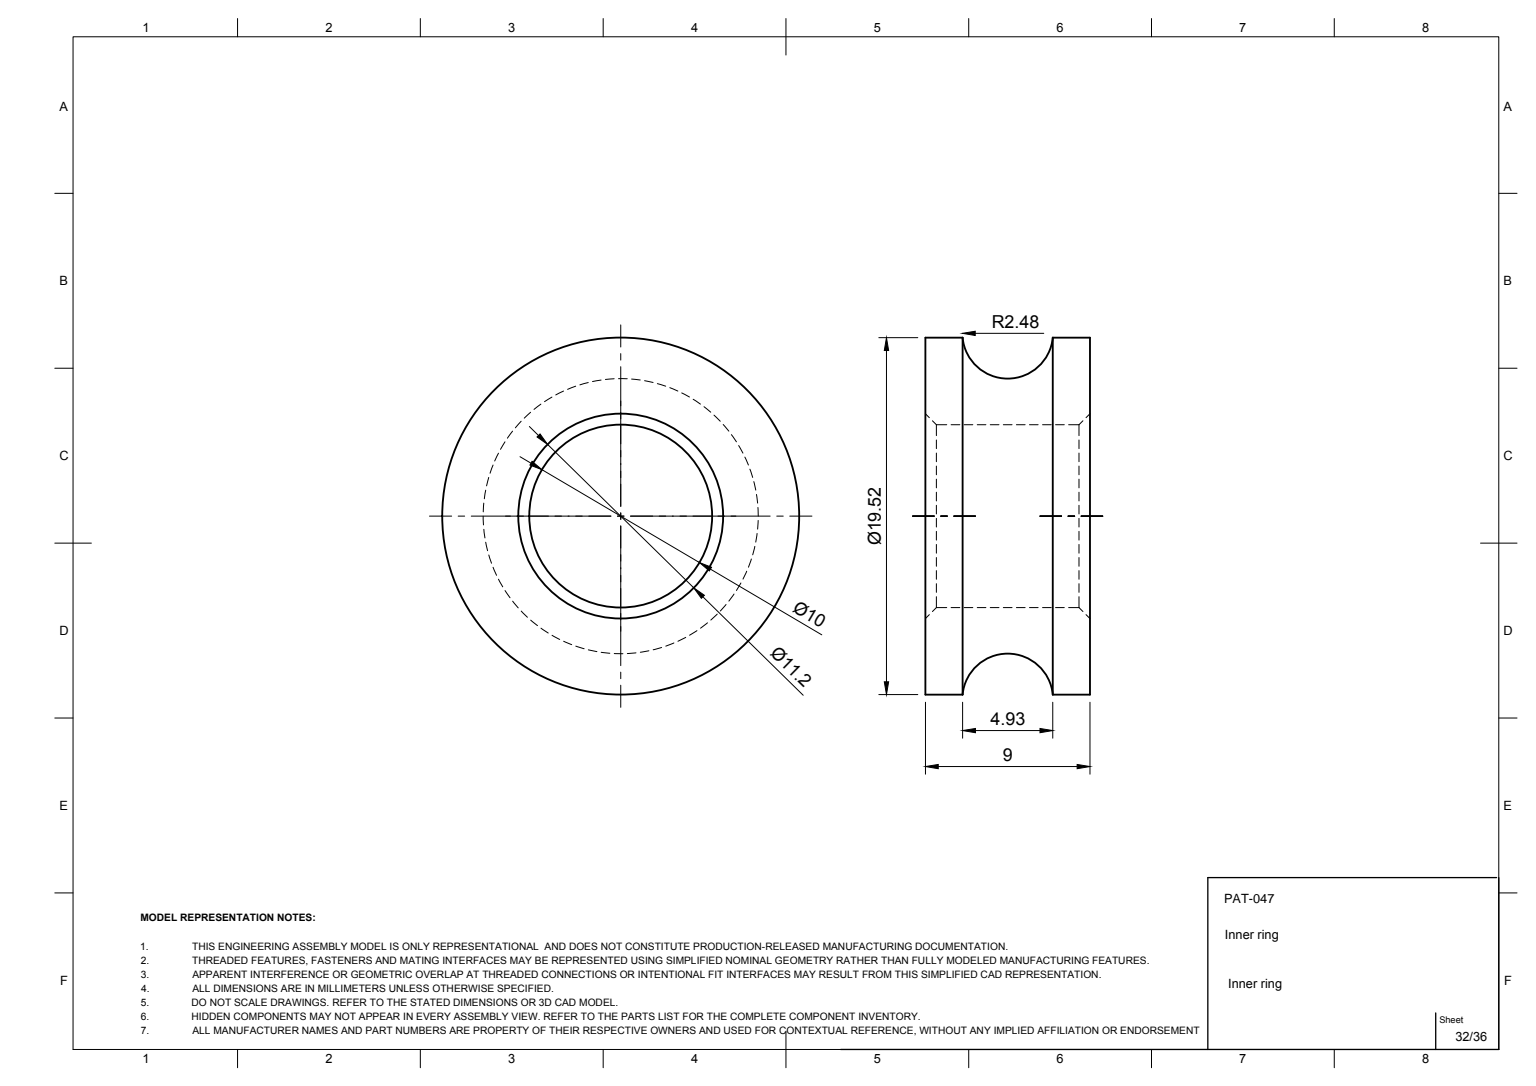
ISO-10303-21;
HEADER;
/* Generated by software containing ST-Developer
 * from STEP Tools, Inc. (www.steptools.com) 
 */

FILE_DESCRIPTION(
/* description */ ('Gravity roller conveyor section'),
/* implementation_level */ '2;1');

FILE_NAME(
/* name */ 'Inner ring.step',
/* time_stamp */ '2026-11-02T07:43:02-08:00',
/* author */ (''),
/* organization */ (''),
/* preprocessor_version */ 'ST-DEVELOPER v20.2',
/* originating_system */ 'Autodesk Translation Framework v15.17.0.0',
/* authorisation */ '');

FILE_SCHEMA (('AUTOMOTIVE_DESIGN { 1 0 10303 214 3 1 1 }'));
ENDSEC;

DATA;
#10=MECHANICAL_DESIGN_GEOMETRIC_PRESENTATION_REPRESENTATION('',(#552),#13821);
#405=TOROIDAL_SURFACE('',#8485,1.,0.247676);
#415=CONICAL_SURFACE('',#8496,0.53,0.785398163397448);
#416=CONICAL_SURFACE('',#8503,0.53,0.785398163397448);
#484=SHAPE_REPRESENTATION_RELATIONSHIP('SRR','None',#14023,#518);
#518=ADVANCED_BREP_SHAPE_REPRESENTATION('',(#592),#13810);
#552=STYLED_ITEM('',(#14191),#592);
#592=MANIFOLD_SOLID_BREP('Body1',#7652);
#678=FACE_BOUND('',#1801,.T.);
#679=FACE_BOUND('',#1804,.T.);
#943=PLANE('',#8498);
#944=PLANE('',#8501);
#1308=FACE_OUTER_BOUND('',#1796,.T.);
#1309=FACE_OUTER_BOUND('',#1797,.T.);
#1310=FACE_OUTER_BOUND('',#1798,.T.);
#1311=FACE_OUTER_BOUND('',#1799,.T.);
#1312=FACE_OUTER_BOUND('',#1800,.T.);
#1313=FACE_OUTER_BOUND('',#1802,.T.);
#1314=FACE_OUTER_BOUND('',#1803,.T.);
#1315=FACE_OUTER_BOUND('',#1805,.T.);
#1796=EDGE_LOOP('',(#6642,#6643,#6644,#6645,#6646,#6647));
#1797=EDGE_LOOP('',(#6648,#6649,#6650,#6651,#6652));
#1798=EDGE_LOOP('',(#6653,#6654,#6655,#6656));
#1799=EDGE_LOOP('',(#6657,#6658,#6659,#6660));
#1800=EDGE_LOOP('',(#6661));
#1801=EDGE_LOOP('',(#6662));
#1802=EDGE_LOOP('',(#6663,#6664,#6665,#6666,#6667));
#1803=EDGE_LOOP('',(#6668));
#1804=EDGE_LOOP('',(#6669));
#1805=EDGE_LOOP('',(#6670,#6671,#6672,#6673));
#2540=LINE('',#12782,#3258);
#2541=LINE('',#12788,#3259);
#2542=LINE('',#12792,#3260);
#2543=LINE('',#12798,#3261);
#2544=LINE('',#12803,#3262);
#3258=VECTOR('',#10307,0.976185);
#3259=VECTOR('',#10314,0.5);
#3260=VECTOR('',#10319,0.53);
#3261=VECTOR('',#10328,0.976185);
#3262=VECTOR('',#10335,0.53);
#3482=CIRCLE('',#8486,0.976185);
#3483=CIRCLE('',#8487,0.976185);
#3484=CIRCLE('',#8488,0.247676);
#3485=CIRCLE('',#8489,0.976185);
#3486=CIRCLE('',#8490,0.976185);
#3487=CIRCLE('',#8492,0.976185);
#3488=CIRCLE('',#8494,0.5);
#3489=CIRCLE('',#8495,0.5);
#3490=CIRCLE('',#8497,0.56);
#3491=CIRCLE('',#8500,0.976185);
#3492=CIRCLE('',#8502,0.56);
#4068=VERTEX_POINT('',#12771);
#4069=VERTEX_POINT('',#12772);
#4070=VERTEX_POINT('',#12775);
#4071=VERTEX_POINT('',#12777);
#4072=VERTEX_POINT('',#12781);
#4073=VERTEX_POINT('',#12785);
#4074=VERTEX_POINT('',#12787);
#4075=VERTEX_POINT('',#12791);
#4076=VERTEX_POINT('',#12796);
#4077=VERTEX_POINT('',#12800);
#4958=EDGE_CURVE('',#4068,#4069,#3482,.T.);
#4959=EDGE_CURVE('',#4069,#4068,#3483,.T.);
#4960=EDGE_CURVE('',#4069,#4070,#3484,.T.);
#4961=EDGE_CURVE('',#4071,#4070,#3485,.T.);
#4962=EDGE_CURVE('',#4070,#4071,#3486,.T.);
#4963=EDGE_CURVE('',#4071,#4072,#2540,.T.);
#4964=EDGE_CURVE('',#4072,#4072,#3487,.T.);
#4965=EDGE_CURVE('',#4073,#4073,#3488,.T.);
#4966=EDGE_CURVE('',#4073,#4074,#2541,.T.);
#4967=EDGE_CURVE('',#4074,#4074,#3489,.T.);
#4968=EDGE_CURVE('',#4074,#4075,#2542,.T.);
#4969=EDGE_CURVE('',#4075,#4075,#3490,.T.);
#4970=EDGE_CURVE('',#4076,#4076,#3491,.T.);
#4971=EDGE_CURVE('',#4076,#4068,#2543,.T.);
#4972=EDGE_CURVE('',#4077,#4077,#3492,.T.);
#4973=EDGE_CURVE('',#4077,#4073,#2544,.T.);
#6642=ORIENTED_EDGE('',*,*,#4958,.F.);
#6643=ORIENTED_EDGE('',*,*,#4959,.F.);
#6644=ORIENTED_EDGE('',*,*,#4960,.T.);
#6645=ORIENTED_EDGE('',*,*,#4961,.F.);
#6646=ORIENTED_EDGE('',*,*,#4962,.F.);
#6647=ORIENTED_EDGE('',*,*,#4960,.F.);
#6648=ORIENTED_EDGE('',*,*,#4961,.T.);
#6649=ORIENTED_EDGE('',*,*,#4962,.T.);
#6650=ORIENTED_EDGE('',*,*,#4963,.T.);
#6651=ORIENTED_EDGE('',*,*,#4964,.T.);
#6652=ORIENTED_EDGE('',*,*,#4963,.F.);
#6653=ORIENTED_EDGE('',*,*,#4965,.T.);
#6654=ORIENTED_EDGE('',*,*,#4966,.T.);
#6655=ORIENTED_EDGE('',*,*,#4967,.F.);
#6656=ORIENTED_EDGE('',*,*,#4966,.F.);
#6657=ORIENTED_EDGE('',*,*,#4967,.T.);
#6658=ORIENTED_EDGE('',*,*,#4968,.T.);
#6659=ORIENTED_EDGE('',*,*,#4969,.F.);
#6660=ORIENTED_EDGE('',*,*,#4968,.F.);
#6661=ORIENTED_EDGE('',*,*,#4964,.F.);
#6662=ORIENTED_EDGE('',*,*,#4969,.T.);
#6663=ORIENTED_EDGE('',*,*,#4970,.F.);
#6664=ORIENTED_EDGE('',*,*,#4971,.T.);
#6665=ORIENTED_EDGE('',*,*,#4958,.T.);
#6666=ORIENTED_EDGE('',*,*,#4959,.T.);
#6667=ORIENTED_EDGE('',*,*,#4971,.F.);
#6668=ORIENTED_EDGE('',*,*,#4970,.T.);
#6669=ORIENTED_EDGE('',*,*,#4972,.F.);
#6670=ORIENTED_EDGE('',*,*,#4972,.T.);
#6671=ORIENTED_EDGE('',*,*,#4973,.T.);
#6672=ORIENTED_EDGE('',*,*,#4965,.F.);
#6673=ORIENTED_EDGE('',*,*,#4973,.F.);
#7182=CYLINDRICAL_SURFACE('',#8491,0.976185);
#7183=CYLINDRICAL_SURFACE('',#8493,0.5);
#7184=CYLINDRICAL_SURFACE('',#8499,0.976185);
#7509=ADVANCED_FACE('',(#1308),#405,.F.);
#7510=ADVANCED_FACE('',(#1309),#7182,.T.);
#7511=ADVANCED_FACE('',(#1310),#7183,.F.);
#7512=ADVANCED_FACE('',(#1311),#415,.F.);
#7513=ADVANCED_FACE('',(#1312,#678),#943,.T.);
#7514=ADVANCED_FACE('',(#1313),#7184,.T.);
#7515=ADVANCED_FACE('',(#1314,#679),#944,.T.);
#7516=ADVANCED_FACE('',(#1315),#416,.F.);
#7652=CLOSED_SHELL('',(#7509,#7510,#7511,#7512,#7513,#7514,#7515,#7516));
#8484=AXIS2_PLACEMENT_3D('',#12769,#10291,#10292);
#8485=AXIS2_PLACEMENT_3D('',#12770,#10293,#10294);
#8486=AXIS2_PLACEMENT_3D('',#12773,#10295,#10296);
#8487=AXIS2_PLACEMENT_3D('',#12774,#10297,#10298);
#8488=AXIS2_PLACEMENT_3D('',#12776,#10299,#10300);
#8489=AXIS2_PLACEMENT_3D('',#12778,#10301,#10302);
#8490=AXIS2_PLACEMENT_3D('',#12779,#10303,#10304);
#8491=AXIS2_PLACEMENT_3D('',#12780,#10305,#10306);
#8492=AXIS2_PLACEMENT_3D('',#12783,#10308,#10309);
#8493=AXIS2_PLACEMENT_3D('',#12784,#10310,#10311);
#8494=AXIS2_PLACEMENT_3D('',#12786,#10312,#10313);
#8495=AXIS2_PLACEMENT_3D('',#12789,#10315,#10316);
#8496=AXIS2_PLACEMENT_3D('',#12790,#10317,#10318);
#8497=AXIS2_PLACEMENT_3D('',#12793,#10320,#10321);
#8498=AXIS2_PLACEMENT_3D('',#12794,#10322,#10323);
#8499=AXIS2_PLACEMENT_3D('',#12795,#10324,#10325);
#8500=AXIS2_PLACEMENT_3D('',#12797,#10326,#10327);
#8501=AXIS2_PLACEMENT_3D('',#12799,#10329,#10330);
#8502=AXIS2_PLACEMENT_3D('',#12801,#10331,#10332);
#8503=AXIS2_PLACEMENT_3D('',#12802,#10333,#10334);
#10291=DIRECTION('axis',(0.,0.,1.));
#10292=DIRECTION('refdir',(1.,0.,0.));
#10293=DIRECTION('center_axis',(0.,-1.,0.));
#10294=DIRECTION('ref_axis',(0.,0.,-1.));
#10295=DIRECTION('center_axis',(0.,-1.,0.));
#10296=DIRECTION('ref_axis',(1.,0.,0.));
#10297=DIRECTION('center_axis',(0.,-1.,0.));
#10298=DIRECTION('ref_axis',(1.,0.,0.));
#10299=DIRECTION('center_axis',(1.,0.,1.22464679914735E-16));
#10300=DIRECTION('ref_axis',(-1.22464679914735E-16,0.,1.));
#10301=DIRECTION('center_axis',(0.,1.,0.));
#10302=DIRECTION('ref_axis',(1.,0.,0.));
#10303=DIRECTION('center_axis',(0.,1.,0.));
#10304=DIRECTION('ref_axis',(1.,0.,0.));
#10305=DIRECTION('center_axis',(0.,-1.,0.));
#10306=DIRECTION('ref_axis',(1.,0.,0.));
#10307=DIRECTION('',(0.,1.,0.));
#10308=DIRECTION('center_axis',(0.,-1.,0.));
#10309=DIRECTION('ref_axis',(1.,0.,0.));
#10310=DIRECTION('center_axis',(0.,-1.,0.));
#10311=DIRECTION('ref_axis',(1.,0.,0.));
#10312=DIRECTION('center_axis',(0.,-1.,0.));
#10313=DIRECTION('ref_axis',(1.,0.,0.));
#10314=DIRECTION('',(0.,1.,0.));
#10315=DIRECTION('center_axis',(0.,-1.,0.));
#10316=DIRECTION('ref_axis',(1.,0.,0.));
#10317=DIRECTION('center_axis',(0.,1.,0.));
#10318=DIRECTION('ref_axis',(1.,0.,0.));
#10319=DIRECTION('',(-0.707106781186547,0.707106781186548,-8.65956056235493E-17));
#10320=DIRECTION('center_axis',(0.,-1.,0.));
#10321=DIRECTION('ref_axis',(1.,0.,0.));
#10322=DIRECTION('center_axis',(0.,1.,0.));
#10323=DIRECTION('ref_axis',(0.,0.,1.));
#10324=DIRECTION('center_axis',(0.,-1.,0.));
#10325=DIRECTION('ref_axis',(1.,0.,0.));
#10326=DIRECTION('center_axis',(0.,-1.,0.));
#10327=DIRECTION('ref_axis',(1.,0.,0.));
#10328=DIRECTION('',(0.,1.,0.));
#10329=DIRECTION('center_axis',(0.,-1.,0.));
#10330=DIRECTION('ref_axis',(0.,0.,-1.));
#10331=DIRECTION('center_axis',(0.,-1.,0.));
#10332=DIRECTION('ref_axis',(1.,0.,0.));
#10333=DIRECTION('center_axis',(0.,-1.,0.));
#10334=DIRECTION('ref_axis',(1.,0.,0.));
#10335=DIRECTION('',(0.707106781186547,0.707106781186548,8.65956056235493E-17));
#12769=CARTESIAN_POINT('',(0.,0.,0.));
#12770=CARTESIAN_POINT('Origin',(0.,0.,0.));
#12771=CARTESIAN_POINT('',(-0.976185,-0.246528389340863,-1.19548183562566E-16));
#12772=CARTESIAN_POINT('',(-1.19548183562566E-16,-0.246528389340863,0.976185));
#12773=CARTESIAN_POINT('Origin',(0.,-0.246528389340863,0.));
#12774=CARTESIAN_POINT('Origin',(0.,-0.246528389340863,0.));
#12775=CARTESIAN_POINT('',(-1.19548183562566E-16,0.246528389340863,0.976185));
#12776=CARTESIAN_POINT('Origin',(-1.22464679914735E-16,0.,1.));
#12777=CARTESIAN_POINT('',(-0.976185,0.246528389340863,1.19548183562566E-16));
#12778=CARTESIAN_POINT('Origin',(0.,0.246528389340863,0.));
#12779=CARTESIAN_POINT('Origin',(0.,0.246528389340863,0.));
#12780=CARTESIAN_POINT('Origin',(0.,0.,0.));
#12781=CARTESIAN_POINT('',(-0.976185,0.45,-1.19548183562566E-16));
#12782=CARTESIAN_POINT('',(-0.976185,0.,-1.19548183562566E-16));
#12783=CARTESIAN_POINT('Origin',(0.,0.45,0.));
#12784=CARTESIAN_POINT('Origin',(0.,0.,0.));
#12785=CARTESIAN_POINT('',(-0.5,-0.39,-6.12323399573677E-17));
#12786=CARTESIAN_POINT('Origin',(0.,-0.39,0.));
#12787=CARTESIAN_POINT('',(-0.5,0.39,-6.12323399573677E-17));
#12788=CARTESIAN_POINT('',(-0.5,0.,-6.12323399573677E-17));
#12789=CARTESIAN_POINT('Origin',(0.,0.39,0.));
#12790=CARTESIAN_POINT('Origin',(0.,0.42,0.));
#12791=CARTESIAN_POINT('',(-0.56,0.45,-6.85802207522518E-17));
#12792=CARTESIAN_POINT('',(-0.53,0.42,-6.49062803548097E-17));
#12793=CARTESIAN_POINT('Origin',(0.,0.45,0.));
#12794=CARTESIAN_POINT('Origin',(0.976185,0.45,0.));
#12795=CARTESIAN_POINT('Origin',(0.,0.,0.));
#12796=CARTESIAN_POINT('',(-0.976185,-0.45,-1.19548183562566E-16));
#12797=CARTESIAN_POINT('Origin',(0.,-0.45,0.));
#12798=CARTESIAN_POINT('',(-0.976185,0.,-1.19548183562566E-16));
#12799=CARTESIAN_POINT('Origin',(0.56,-0.45,0.));
#12800=CARTESIAN_POINT('',(-0.56,-0.45,-6.85802207522518E-17));
#12801=CARTESIAN_POINT('Origin',(0.,-0.45,0.));
#12802=CARTESIAN_POINT('Origin',(0.,-0.42,0.));
#12803=CARTESIAN_POINT('',(-0.53,-0.42,-6.49062803548097E-17));
#13771=UNCERTAINTY_MEASURE_WITH_UNIT(LENGTH_MEASURE(0.001),#13822,
'DISTANCE_ACCURACY_VALUE',
'Maximum model space distance between geometric entities at asserted c
onnectivities');
#13782=UNCERTAINTY_MEASURE_WITH_UNIT(LENGTH_MEASURE(0.001),#13822,
'DISTANCE_ACCURACY_VALUE',
'Maximum model space distance between geometric entities at asserted c
onnectivities');
#13810=(
GEOMETRIC_REPRESENTATION_CONTEXT(3)
GLOBAL_UNCERTAINTY_ASSIGNED_CONTEXT((#13771))
GLOBAL_UNIT_ASSIGNED_CONTEXT((#13822,#13824,#13825))
REPRESENTATION_CONTEXT('','3D')
);
#13821=(
GEOMETRIC_REPRESENTATION_CONTEXT(3)
GLOBAL_UNCERTAINTY_ASSIGNED_CONTEXT((#13782))
GLOBAL_UNIT_ASSIGNED_CONTEXT((#13822,#13824,#13825))
REPRESENTATION_CONTEXT('','3D')
);
#13822=(
LENGTH_UNIT()
NAMED_UNIT(*)
SI_UNIT(.CENTI.,.METRE.)
);
#13824=(
NAMED_UNIT(*)
PLANE_ANGLE_UNIT()
SI_UNIT($,.RADIAN.)
);
#13825=(
NAMED_UNIT(*)
SI_UNIT($,.STERADIAN.)
SOLID_ANGLE_UNIT()
);
#13853=SHAPE_DEFINITION_REPRESENTATION(#13891,#14023);
#13891=PRODUCT_DEFINITION_SHAPE('',$,#14062);
#14023=SHAPE_REPRESENTATION('',(#8484),#13810);
#14034=PRODUCT_DEFINITION_CONTEXT('part definition',#14150,'design');
#14062=PRODUCT_DEFINITION('Inner ring','Inner ring',#14100,#14034);
#14100=PRODUCT_DEFINITION_FORMATION('',$,#14179);
#14150=APPLICATION_CONTEXT(
'Core Data for Automotive Mechanical Design Process');
#14151=PRODUCT_CONTEXT('part definition',#14150,'mechanical');
#14179=PRODUCT('Inner ring','Inner ring','Inner ring',(#14151));
#14191=PRESENTATION_STYLE_ASSIGNMENT((#14196));
#14196=SURFACE_STYLE_USAGE(.BOTH.,#14201);
#14201=SURFACE_SIDE_STYLE('',(#14206));
#14206=SURFACE_STYLE_FILL_AREA(#14211);
#14211=FILL_AREA_STYLE('CAD Library Painted - Steel gray',(#14216));
#14216=FILL_AREA_STYLE_COLOUR('CAD Library Painted - Steel gray',#14221);
#14221=COLOUR_RGB('CAD Library Painted - Steel gray',0.592156862745098,
0.631372549019608,0.67843137254902);
ENDSEC;
END-ISO-10303-21;
